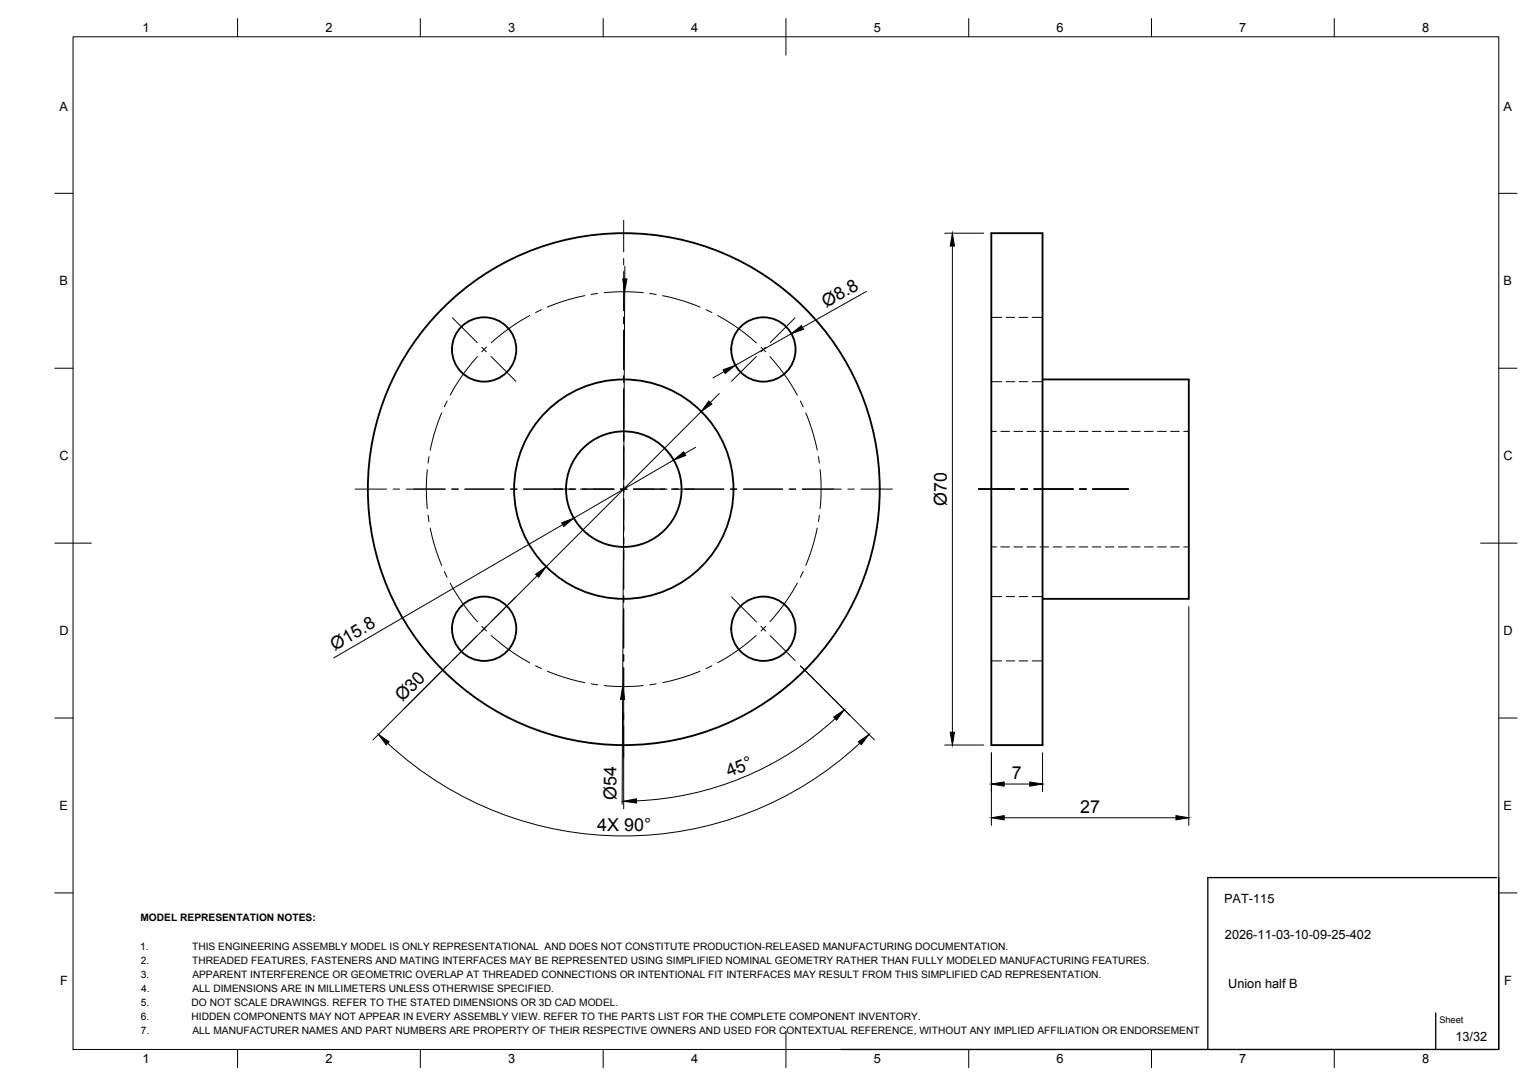
ISO-10303-21;
HEADER;
/* Generated by software containing ST-Developer
 * from STEP Tools, Inc. (www.steptools.com) 
 */

FILE_DESCRIPTION(
/* description */ ('Union bypass pipe loop'),
/* implementation_level */ '2;1');

FILE_NAME(
/* name */ 'Union half B.step',
/* time_stamp */ '2026-10-27T21:00:29-07:00',
/* author */ (''),
/* organization */ (''),
/* preprocessor_version */ 'ST-DEVELOPER v20.2',
/* originating_system */ 'Autodesk Translation Framework v15.17.0.0',
/* authorisation */ '');

FILE_SCHEMA (('AUTOMOTIVE_DESIGN { 1 0 10303 214 3 1 1 }'));
ENDSEC;

DATA;
#10=MECHANICAL_DESIGN_GEOMETRIC_PRESENTATION_REPRESENTATION('',(#467),#10095);
#403=SHAPE_REPRESENTATION_RELATIONSHIP('SRR','None',#10272,#435);
#435=ADVANCED_BREP_SHAPE_REPRESENTATION('',(#497),#10084);
#467=STYLED_ITEM('',(#10493),#497);
#497=MANIFOLD_SOLID_BREP('Body1',#5540);
#610=FACE_BOUND('',#1496,.T.);
#611=FACE_BOUND('',#1497,.T.);
#612=FACE_BOUND('',#1498,.T.);
#613=FACE_BOUND('',#1499,.T.);
#614=FACE_BOUND('',#1500,.T.);
#615=FACE_BOUND('',#1505,.T.);
#616=FACE_BOUND('',#1507,.T.);
#617=FACE_BOUND('',#1508,.T.);
#618=FACE_BOUND('',#1509,.T.);
#619=FACE_BOUND('',#1510,.T.);
#620=FACE_BOUND('',#1511,.T.);
#757=PLANE('',#6413);
#758=PLANE('',#6423);
#759=PLANE('',#6424);
#1060=FACE_OUTER_BOUND('',#1491,.T.);
#1061=FACE_OUTER_BOUND('',#1492,.T.);
#1062=FACE_OUTER_BOUND('',#1493,.T.);
#1063=FACE_OUTER_BOUND('',#1494,.T.);
#1064=FACE_OUTER_BOUND('',#1495,.T.);
#1065=FACE_OUTER_BOUND('',#1501,.T.);
#1066=FACE_OUTER_BOUND('',#1502,.T.);
#1067=FACE_OUTER_BOUND('',#1503,.T.);
#1068=FACE_OUTER_BOUND('',#1504,.T.);
#1069=FACE_OUTER_BOUND('',#1506,.T.);
#1491=EDGE_LOOP('',(#4642,#4643,#4644,#4645));
#1492=EDGE_LOOP('',(#4646,#4647,#4648,#4649));
#1493=EDGE_LOOP('',(#4650,#4651,#4652,#4653));
#1494=EDGE_LOOP('',(#4654,#4655,#4656,#4657));
#1495=EDGE_LOOP('',(#4658));
#1496=EDGE_LOOP('',(#4659));
#1497=EDGE_LOOP('',(#4660));
#1498=EDGE_LOOP('',(#4661));
#1499=EDGE_LOOP('',(#4662));
#1500=EDGE_LOOP('',(#4663));
#1501=EDGE_LOOP('',(#4664,#4665,#4666,#4667));
#1502=EDGE_LOOP('',(#4668,#4669,#4670,#4671));
#1503=EDGE_LOOP('',(#4672,#4673,#4674,#4675));
#1504=EDGE_LOOP('',(#4676));
#1505=EDGE_LOOP('',(#4677));
#1506=EDGE_LOOP('',(#4678));
#1507=EDGE_LOOP('',(#4679));
#1508=EDGE_LOOP('',(#4680));
#1509=EDGE_LOOP('',(#4681));
#1510=EDGE_LOOP('',(#4682));
#1511=EDGE_LOOP('',(#4683));
#1853=LINE('',#9485,#2229);
#1854=LINE('',#9491,#2230);
#1855=LINE('',#9497,#2231);
#1856=LINE('',#9503,#2232);
#1857=LINE('',#9512,#2233);
#1858=LINE('',#9518,#2234);
#1859=LINE('',#9523,#2235);
#2229=VECTOR('',#7845,0.44);
#2230=VECTOR('',#7852,0.44);
#2231=VECTOR('',#7859,0.44);
#2232=VECTOR('',#7866,0.44);
#2233=VECTOR('',#7877,3.5);
#2234=VECTOR('',#7884,0.79);
#2235=VECTOR('',#7891,1.5);
#2569=CIRCLE('',#6402,0.44);
#2570=CIRCLE('',#6403,0.44);
#2571=CIRCLE('',#6405,0.44);
#2572=CIRCLE('',#6406,0.44);
#2573=CIRCLE('',#6408,0.44);
#2574=CIRCLE('',#6409,0.44);
#2575=CIRCLE('',#6411,0.44);
#2576=CIRCLE('',#6412,0.44);
#2577=CIRCLE('',#6414,3.5);
#2578=CIRCLE('',#6415,1.5);
#2579=CIRCLE('',#6417,3.5);
#2580=CIRCLE('',#6419,0.79);
#2581=CIRCLE('',#6420,0.79);
#2582=CIRCLE('',#6422,1.5);
#2926=VERTEX_POINT('',#9482);
#2927=VERTEX_POINT('',#9484);
#2928=VERTEX_POINT('',#9488);
#2929=VERTEX_POINT('',#9490);
#2930=VERTEX_POINT('',#9494);
#2931=VERTEX_POINT('',#9496);
#2932=VERTEX_POINT('',#9500);
#2933=VERTEX_POINT('',#9502);
#2934=VERTEX_POINT('',#9506);
#2935=VERTEX_POINT('',#9508);
#2936=VERTEX_POINT('',#9511);
#2937=VERTEX_POINT('',#9515);
#2938=VERTEX_POINT('',#9517);
#2939=VERTEX_POINT('',#9521);
#3519=EDGE_CURVE('',#2926,#2926,#2569,.T.);
#3520=EDGE_CURVE('',#2926,#2927,#1853,.T.);
#3521=EDGE_CURVE('',#2927,#2927,#2570,.T.);
#3522=EDGE_CURVE('',#2928,#2928,#2571,.T.);
#3523=EDGE_CURVE('',#2928,#2929,#1854,.T.);
#3524=EDGE_CURVE('',#2929,#2929,#2572,.T.);
#3525=EDGE_CURVE('',#2930,#2930,#2573,.T.);
#3526=EDGE_CURVE('',#2930,#2931,#1855,.T.);
#3527=EDGE_CURVE('',#2931,#2931,#2574,.T.);
#3528=EDGE_CURVE('',#2932,#2932,#2575,.T.);
#3529=EDGE_CURVE('',#2932,#2933,#1856,.T.);
#3530=EDGE_CURVE('',#2933,#2933,#2576,.T.);
#3531=EDGE_CURVE('',#2934,#2934,#2577,.T.);
#3532=EDGE_CURVE('',#2935,#2935,#2578,.T.);
#3533=EDGE_CURVE('',#2934,#2936,#1857,.T.);
#3534=EDGE_CURVE('',#2936,#2936,#2579,.T.);
#3535=EDGE_CURVE('',#2937,#2937,#2580,.T.);
#3536=EDGE_CURVE('',#2937,#2938,#1858,.T.);
#3537=EDGE_CURVE('',#2938,#2938,#2581,.T.);
#3538=EDGE_CURVE('',#2939,#2939,#2582,.T.);
#3539=EDGE_CURVE('',#2939,#2935,#1859,.T.);
#4642=ORIENTED_EDGE('',*,*,#3519,.F.);
#4643=ORIENTED_EDGE('',*,*,#3520,.T.);
#4644=ORIENTED_EDGE('',*,*,#3521,.F.);
#4645=ORIENTED_EDGE('',*,*,#3520,.F.);
#4646=ORIENTED_EDGE('',*,*,#3522,.F.);
#4647=ORIENTED_EDGE('',*,*,#3523,.T.);
#4648=ORIENTED_EDGE('',*,*,#3524,.F.);
#4649=ORIENTED_EDGE('',*,*,#3523,.F.);
#4650=ORIENTED_EDGE('',*,*,#3525,.F.);
#4651=ORIENTED_EDGE('',*,*,#3526,.T.);
#4652=ORIENTED_EDGE('',*,*,#3527,.F.);
#4653=ORIENTED_EDGE('',*,*,#3526,.F.);
#4654=ORIENTED_EDGE('',*,*,#3528,.F.);
#4655=ORIENTED_EDGE('',*,*,#3529,.T.);
#4656=ORIENTED_EDGE('',*,*,#3530,.F.);
#4657=ORIENTED_EDGE('',*,*,#3529,.F.);
#4658=ORIENTED_EDGE('',*,*,#3531,.T.);
#4659=ORIENTED_EDGE('',*,*,#3532,.F.);
#4660=ORIENTED_EDGE('',*,*,#3530,.T.);
#4661=ORIENTED_EDGE('',*,*,#3527,.T.);
#4662=ORIENTED_EDGE('',*,*,#3524,.T.);
#4663=ORIENTED_EDGE('',*,*,#3521,.T.);
#4664=ORIENTED_EDGE('',*,*,#3531,.F.);
#4665=ORIENTED_EDGE('',*,*,#3533,.T.);
#4666=ORIENTED_EDGE('',*,*,#3534,.T.);
#4667=ORIENTED_EDGE('',*,*,#3533,.F.);
#4668=ORIENTED_EDGE('',*,*,#3535,.F.);
#4669=ORIENTED_EDGE('',*,*,#3536,.T.);
#4670=ORIENTED_EDGE('',*,*,#3537,.T.);
#4671=ORIENTED_EDGE('',*,*,#3536,.F.);
#4672=ORIENTED_EDGE('',*,*,#3538,.F.);
#4673=ORIENTED_EDGE('',*,*,#3539,.T.);
#4674=ORIENTED_EDGE('',*,*,#3532,.T.);
#4675=ORIENTED_EDGE('',*,*,#3539,.F.);
#4676=ORIENTED_EDGE('',*,*,#3538,.T.);
#4677=ORIENTED_EDGE('',*,*,#3535,.T.);
#4678=ORIENTED_EDGE('',*,*,#3534,.F.);
#4679=ORIENTED_EDGE('',*,*,#3537,.F.);
#4680=ORIENTED_EDGE('',*,*,#3528,.T.);
#4681=ORIENTED_EDGE('',*,*,#3525,.T.);
#4682=ORIENTED_EDGE('',*,*,#3522,.T.);
#4683=ORIENTED_EDGE('',*,*,#3519,.T.);
#5165=CYLINDRICAL_SURFACE('',#6401,0.44);
#5166=CYLINDRICAL_SURFACE('',#6404,0.44);
#5167=CYLINDRICAL_SURFACE('',#6407,0.44);
#5168=CYLINDRICAL_SURFACE('',#6410,0.44);
#5169=CYLINDRICAL_SURFACE('',#6416,3.5);
#5170=CYLINDRICAL_SURFACE('',#6418,0.79);
#5171=CYLINDRICAL_SURFACE('',#6421,1.5);
#5409=ADVANCED_FACE('',(#1060),#5165,.F.);
#5410=ADVANCED_FACE('',(#1061),#5166,.F.);
#5411=ADVANCED_FACE('',(#1062),#5167,.F.);
#5412=ADVANCED_FACE('',(#1063),#5168,.F.);
#5413=ADVANCED_FACE('',(#1064,#610,#611,#612,#613,#614),#757,.T.);
#5414=ADVANCED_FACE('',(#1065),#5169,.T.);
#5415=ADVANCED_FACE('',(#1066),#5170,.F.);
#5416=ADVANCED_FACE('',(#1067),#5171,.T.);
#5417=ADVANCED_FACE('',(#1068,#615),#758,.T.);
#5418=ADVANCED_FACE('',(#1069,#616,#617,#618,#619,#620),#759,.F.);
#5540=CLOSED_SHELL('',(#5409,#5410,#5411,#5412,#5413,#5414,#5415,#5416,
#5417,#5418));
#6400=AXIS2_PLACEMENT_3D('',#9480,#7839,#7840);
#6401=AXIS2_PLACEMENT_3D('',#9481,#7841,#7842);
#6402=AXIS2_PLACEMENT_3D('',#9483,#7843,#7844);
#6403=AXIS2_PLACEMENT_3D('',#9486,#7846,#7847);
#6404=AXIS2_PLACEMENT_3D('',#9487,#7848,#7849);
#6405=AXIS2_PLACEMENT_3D('',#9489,#7850,#7851);
#6406=AXIS2_PLACEMENT_3D('',#9492,#7853,#7854);
#6407=AXIS2_PLACEMENT_3D('',#9493,#7855,#7856);
#6408=AXIS2_PLACEMENT_3D('',#9495,#7857,#7858);
#6409=AXIS2_PLACEMENT_3D('',#9498,#7860,#7861);
#6410=AXIS2_PLACEMENT_3D('',#9499,#7862,#7863);
#6411=AXIS2_PLACEMENT_3D('',#9501,#7864,#7865);
#6412=AXIS2_PLACEMENT_3D('',#9504,#7867,#7868);
#6413=AXIS2_PLACEMENT_3D('',#9505,#7869,#7870);
#6414=AXIS2_PLACEMENT_3D('',#9507,#7871,#7872);
#6415=AXIS2_PLACEMENT_3D('',#9509,#7873,#7874);
#6416=AXIS2_PLACEMENT_3D('',#9510,#7875,#7876);
#6417=AXIS2_PLACEMENT_3D('',#9513,#7878,#7879);
#6418=AXIS2_PLACEMENT_3D('',#9514,#7880,#7881);
#6419=AXIS2_PLACEMENT_3D('',#9516,#7882,#7883);
#6420=AXIS2_PLACEMENT_3D('',#9519,#7885,#7886);
#6421=AXIS2_PLACEMENT_3D('',#9520,#7887,#7888);
#6422=AXIS2_PLACEMENT_3D('',#9522,#7889,#7890);
#6423=AXIS2_PLACEMENT_3D('',#9524,#7892,#7893);
#6424=AXIS2_PLACEMENT_3D('',#9525,#7894,#7895);
#7839=DIRECTION('axis',(0.,0.,1.));
#7840=DIRECTION('refdir',(1.,0.,0.));
#7841=DIRECTION('center_axis',(1.,0.,0.));
#7842=DIRECTION('ref_axis',(0.,0.,-1.));
#7843=DIRECTION('center_axis',(1.,0.,0.));
#7844=DIRECTION('ref_axis',(0.,0.,-1.));
#7845=DIRECTION('',(1.,0.,0.));
#7846=DIRECTION('center_axis',(-1.,0.,0.));
#7847=DIRECTION('ref_axis',(0.,0.,-1.));
#7848=DIRECTION('center_axis',(1.,0.,0.));
#7849=DIRECTION('ref_axis',(0.,0.,-1.));
#7850=DIRECTION('center_axis',(1.,0.,0.));
#7851=DIRECTION('ref_axis',(0.,0.,-1.));
#7852=DIRECTION('',(1.,0.,0.));
#7853=DIRECTION('center_axis',(-1.,0.,0.));
#7854=DIRECTION('ref_axis',(0.,0.,-1.));
#7855=DIRECTION('center_axis',(1.,0.,0.));
#7856=DIRECTION('ref_axis',(0.,0.,-1.));
#7857=DIRECTION('center_axis',(1.,0.,0.));
#7858=DIRECTION('ref_axis',(0.,0.,-1.));
#7859=DIRECTION('',(1.,0.,0.));
#7860=DIRECTION('center_axis',(-1.,0.,0.));
#7861=DIRECTION('ref_axis',(0.,0.,-1.));
#7862=DIRECTION('center_axis',(1.,0.,0.));
#7863=DIRECTION('ref_axis',(0.,0.,-1.));
#7864=DIRECTION('center_axis',(1.,0.,0.));
#7865=DIRECTION('ref_axis',(0.,0.,-1.));
#7866=DIRECTION('',(1.,0.,0.));
#7867=DIRECTION('center_axis',(-1.,0.,0.));
#7868=DIRECTION('ref_axis',(0.,0.,-1.));
#7869=DIRECTION('center_axis',(1.,0.,0.));
#7870=DIRECTION('ref_axis',(0.,0.,-1.));
#7871=DIRECTION('center_axis',(1.,0.,0.));
#7872=DIRECTION('ref_axis',(0.,0.,-1.));
#7873=DIRECTION('center_axis',(1.,0.,0.));
#7874=DIRECTION('ref_axis',(0.,0.,-1.));
#7875=DIRECTION('center_axis',(1.,0.,0.));
#7876=DIRECTION('ref_axis',(0.,0.,-1.));
#7877=DIRECTION('',(-1.,0.,0.));
#7878=DIRECTION('center_axis',(1.,0.,0.));
#7879=DIRECTION('ref_axis',(0.,0.,-1.));
#7880=DIRECTION('center_axis',(1.,0.,0.));
#7881=DIRECTION('ref_axis',(0.,0.,-1.));
#7882=DIRECTION('center_axis',(-1.,0.,0.));
#7883=DIRECTION('ref_axis',(0.,0.,-1.));
#7884=DIRECTION('',(-1.,0.,0.));
#7885=DIRECTION('center_axis',(-1.,0.,0.));
#7886=DIRECTION('ref_axis',(0.,0.,-1.));
#7887=DIRECTION('center_axis',(1.,0.,0.));
#7888=DIRECTION('ref_axis',(0.,0.,-1.));
#7889=DIRECTION('center_axis',(1.,0.,0.));
#7890=DIRECTION('ref_axis',(0.,0.,-1.));
#7891=DIRECTION('',(-1.,0.,0.));
#7892=DIRECTION('center_axis',(1.,0.,0.));
#7893=DIRECTION('ref_axis',(0.,0.,-1.));
#7894=DIRECTION('center_axis',(1.,0.,0.));
#7895=DIRECTION('ref_axis',(0.,0.,-1.));
#9480=CARTESIAN_POINT('',(0.,0.,0.));
#9481=CARTESIAN_POINT('Origin',(0.,-1.90918830920368,4.09081169079632));
#9482=CARTESIAN_POINT('',(0.1,-1.90918830920368,4.53081169079632));
#9483=CARTESIAN_POINT('Origin',(0.1,-1.90918830920368,4.09081169079632));
#9484=CARTESIAN_POINT('',(0.8,-1.90918830920368,4.53081169079632));
#9485=CARTESIAN_POINT('',(0.,-1.90918830920368,4.53081169079632));
#9486=CARTESIAN_POINT('Origin',(0.8,-1.90918830920368,4.09081169079632));
#9487=CARTESIAN_POINT('Origin',(0.,-1.90918830920368,7.90918830920368));
#9488=CARTESIAN_POINT('',(0.1,-1.90918830920368,8.34918830920368));
#9489=CARTESIAN_POINT('Origin',(0.1,-1.90918830920368,7.90918830920368));
#9490=CARTESIAN_POINT('',(0.8,-1.90918830920368,8.34918830920368));
#9491=CARTESIAN_POINT('',(0.,-1.90918830920368,8.34918830920368));
#9492=CARTESIAN_POINT('Origin',(0.8,-1.90918830920368,7.90918830920368));
#9493=CARTESIAN_POINT('Origin',(0.,1.90918830920368,7.90918830920368));
#9494=CARTESIAN_POINT('',(0.1,1.90918830920368,8.34918830920368));
#9495=CARTESIAN_POINT('Origin',(0.1,1.90918830920368,7.90918830920368));
#9496=CARTESIAN_POINT('',(0.8,1.90918830920368,8.34918830920368));
#9497=CARTESIAN_POINT('',(0.,1.90918830920368,8.34918830920368));
#9498=CARTESIAN_POINT('Origin',(0.8,1.90918830920368,7.90918830920368));
#9499=CARTESIAN_POINT('Origin',(0.,1.90918830920368,4.09081169079632));
#9500=CARTESIAN_POINT('',(0.1,1.90918830920368,4.53081169079632));
#9501=CARTESIAN_POINT('Origin',(0.1,1.90918830920368,4.09081169079632));
#9502=CARTESIAN_POINT('',(0.8,1.90918830920368,4.53081169079632));
#9503=CARTESIAN_POINT('',(0.,1.90918830920368,4.53081169079632));
#9504=CARTESIAN_POINT('Origin',(0.8,1.90918830920368,4.09081169079632));
#9505=CARTESIAN_POINT('Origin',(0.8,0.,6.));
#9506=CARTESIAN_POINT('',(0.8,-4.28626379701574E-16,9.5));
#9507=CARTESIAN_POINT('Origin',(0.8,0.,6.));
#9508=CARTESIAN_POINT('',(0.8,-1.83697019872103E-16,7.5));
#9509=CARTESIAN_POINT('Origin',(0.8,0.,6.));
#9510=CARTESIAN_POINT('Origin',(0.1,0.,6.));
#9511=CARTESIAN_POINT('',(0.1,-4.28626379701574E-16,9.5));
#9512=CARTESIAN_POINT('',(0.1,-4.28626379701574E-16,9.5));
#9513=CARTESIAN_POINT('Origin',(0.1,0.,6.));
#9514=CARTESIAN_POINT('Origin',(0.1,0.,6.));
#9515=CARTESIAN_POINT('',(2.8,-9.67470971326409E-17,6.79));
#9516=CARTESIAN_POINT('Origin',(2.8,0.,6.));
#9517=CARTESIAN_POINT('',(0.1,-9.67470971326409E-17,6.79));
#9518=CARTESIAN_POINT('',(0.1,-9.67470971326409E-17,6.79));
#9519=CARTESIAN_POINT('Origin',(0.1,0.,6.));
#9520=CARTESIAN_POINT('Origin',(0.1,0.,6.));
#9521=CARTESIAN_POINT('',(2.8,-1.83697019872103E-16,7.5));
#9522=CARTESIAN_POINT('Origin',(2.8,0.,6.));
#9523=CARTESIAN_POINT('',(0.1,-1.83697019872103E-16,7.5));
#9524=CARTESIAN_POINT('Origin',(2.8,0.,6.));
#9525=CARTESIAN_POINT('Origin',(0.1,0.,6.));
#10047=UNCERTAINTY_MEASURE_WITH_UNIT(LENGTH_MEASURE(0.001),#10096,
'DISTANCE_ACCURACY_VALUE',
'Maximum model space distance between geometric entities at asserted c
onnectivities');
#10058=UNCERTAINTY_MEASURE_WITH_UNIT(LENGTH_MEASURE(0.001),#10096,
'DISTANCE_ACCURACY_VALUE',
'Maximum model space distance between geometric entities at asserted c
onnectivities');
#10084=(
GEOMETRIC_REPRESENTATION_CONTEXT(3)
GLOBAL_UNCERTAINTY_ASSIGNED_CONTEXT((#10047))
GLOBAL_UNIT_ASSIGNED_CONTEXT((#10096,#10098,#10099))
REPRESENTATION_CONTEXT('','3D')
);
#10095=(
GEOMETRIC_REPRESENTATION_CONTEXT(3)
GLOBAL_UNCERTAINTY_ASSIGNED_CONTEXT((#10058))
GLOBAL_UNIT_ASSIGNED_CONTEXT((#10096,#10098,#10099))
REPRESENTATION_CONTEXT('','3D')
);
#10096=(
LENGTH_UNIT()
NAMED_UNIT(*)
SI_UNIT(.CENTI.,.METRE.)
);
#10098=(
NAMED_UNIT(*)
PLANE_ANGLE_UNIT()
SI_UNIT($,.RADIAN.)
);
#10099=(
NAMED_UNIT(*)
SI_UNIT($,.STERADIAN.)
SOLID_ANGLE_UNIT()
);
#10125=SHAPE_DEFINITION_REPRESENTATION(#10196,#10272);
#10196=PRODUCT_DEFINITION_SHAPE('',$,#10309);
#10272=SHAPE_REPRESENTATION('',(#6400),#10084);
#10283=PRODUCT_DEFINITION_CONTEXT('part definition',#10393,'design');
#10309=PRODUCT_DEFINITION('Union half B','Union half B',#10345,#10283);
#10345=PRODUCT_DEFINITION_FORMATION('',$,#10420);
#10393=APPLICATION_CONTEXT(
'Core Data for Automotive Mechanical Design Process');
#10394=PRODUCT_CONTEXT('part definition',#10393,'mechanical');
#10420=PRODUCT('Union half B','Union half B','Union half B',(#10394));
#10487=COLOUR_RGB('Sky Blue',0.24,0.69,0.87);
#10488=FILL_AREA_STYLE_COLOUR('',#10487);
#10489=FILL_AREA_STYLE('',(#10488));
#10490=SURFACE_STYLE_FILL_AREA(#10489);
#10491=SURFACE_SIDE_STYLE('',(#10490));
#10492=SURFACE_STYLE_USAGE(.BOTH.,#10491);
#10493=PRESENTATION_STYLE_ASSIGNMENT((#10492));
ENDSEC;
END-ISO-10303-21;
